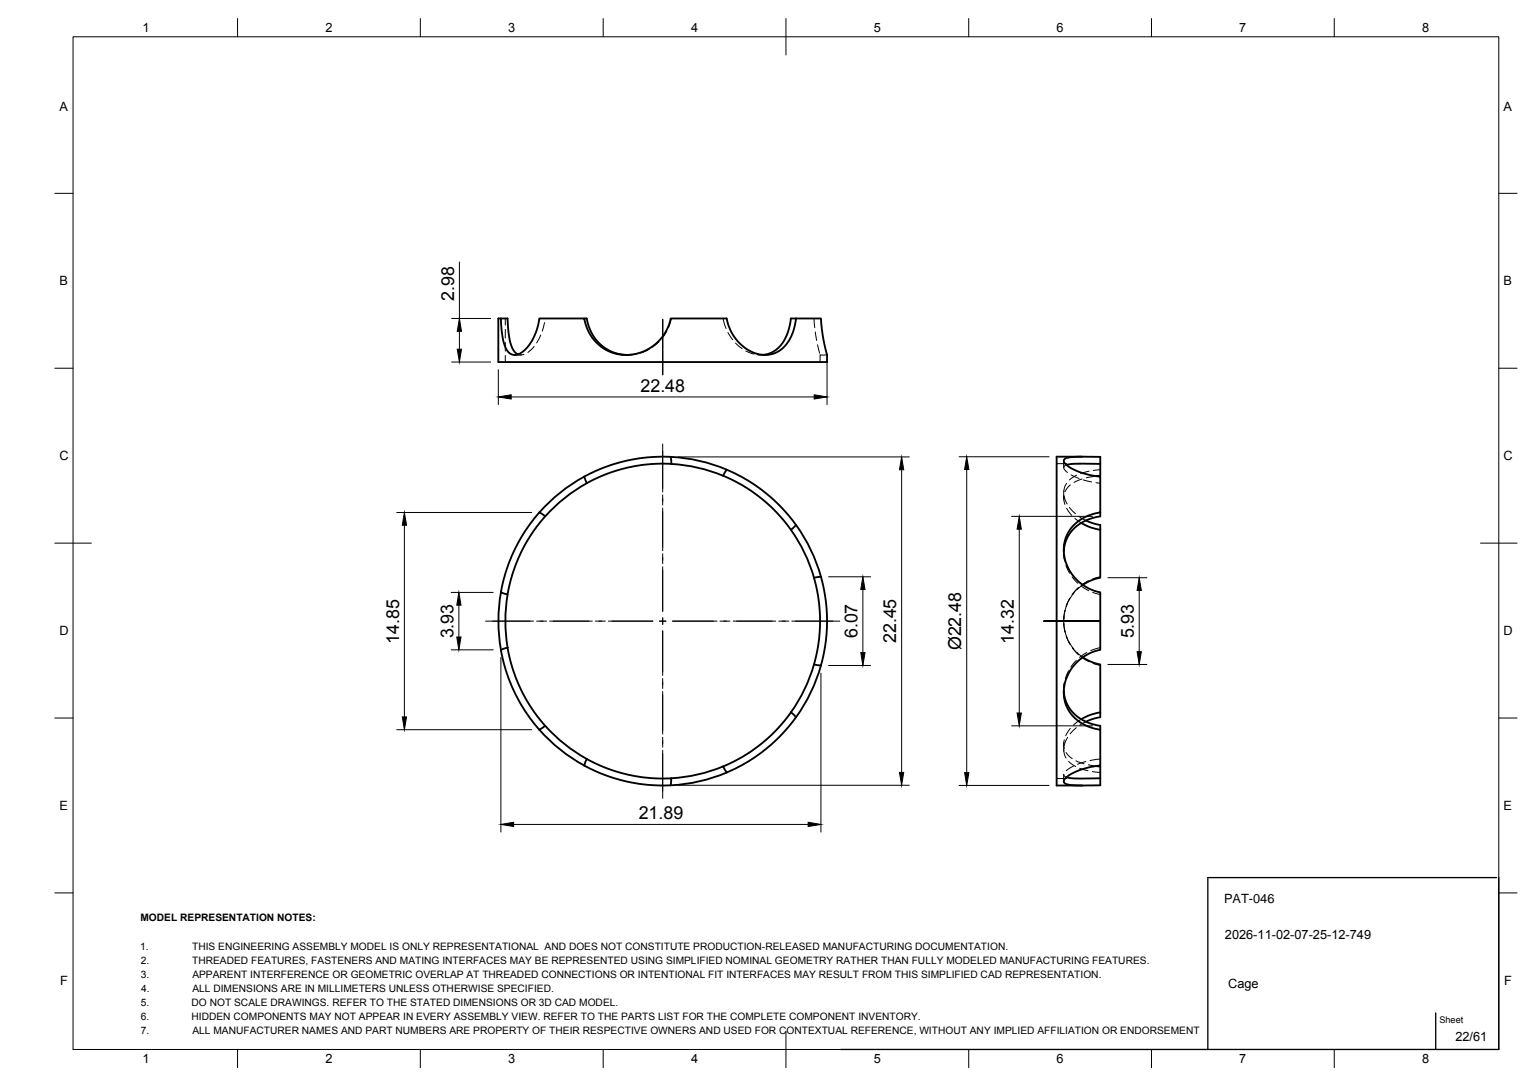
ISO-10303-21;
HEADER;
/* Generated by software containing ST-Developer
 * from STEP Tools, Inc. (www.steptools.com) 
 */

FILE_DESCRIPTION(
/* description */ ('Gear mesh backlash fixture'),
/* implementation_level */ '2;1');

FILE_NAME(
/* name */ 'Cage.step',
/* time_stamp */ '2026-10-28T03:26:00-07:00',
/* author */ (''),
/* organization */ (''),
/* preprocessor_version */ 'ST-DEVELOPER v20.2',
/* originating_system */ 'Autodesk Translation Framework v15.17.0.0',
/* authorisation */ '');

FILE_SCHEMA (('AUTOMOTIVE_DESIGN { 1 0 10303 214 3 1 1 }'));
ENDSEC;

DATA;
#10=MECHANICAL_DESIGN_GEOMETRIC_PRESENTATION_REPRESENTATION('',(#1037),#57900);
#736=SPHERICAL_SURFACE('',#14553,0.309556);
#737=SPHERICAL_SURFACE('',#14569,0.309556);
#738=SPHERICAL_SURFACE('',#14574,0.309556);
#739=SPHERICAL_SURFACE('',#14580,0.309556);
#740=SPHERICAL_SURFACE('',#14585,0.309556);
#741=SPHERICAL_SURFACE('',#14590,0.309556);
#742=SPHERICAL_SURFACE('',#14598,0.309556);
#791=B_SPLINE_CURVE_WITH_KNOTS('',3,(#20144,#20145,#20146,#20147,#20148,
#20149,#20150,#20151,#20152,#20153,#20154,#20155,#20156,#20157,#20158,#20159,
#20160,#20161,#20162,#20163,#20164,#20165),.UNSPECIFIED.,.F.,.F.,(4,2,2,
2,2,2,2,2,2,2,4),(0.0591825211272536,0.157966726598481,0.236950089897721,
0.315933453196962,0.391576304923761,0.46721915665056,0.54286200837736,0.618504860104159,
0.697488223403399,0.77647158670264,0.875255792173867),.UNSPECIFIED.);
#792=B_SPLINE_CURVE_WITH_KNOTS('',3,(#20169,#20170,#20171,#20172,#20173,
#20174,#20175,#20176,#20177,#20178,#20179,#20180,#20181,#20182,#20183,#20184,
#20185,#20186,#20187,#20188,#20189,#20190),.UNSPECIFIED.,.F.,.F.,(4,2,2,
2,2,2,2,2,2,2,4),(0.0581119756758434,0.106553146291161,0.213106292582322,
0.30849933801665,0.386091982889075,0.4636846277615,0.541277272633925,0.61886991750635,
0.714262962940678,0.820816109231839,0.869257279847157),.UNSPECIFIED.);
#793=B_SPLINE_CURVE_WITH_KNOTS('',3,(#20196,#20197,#20198,#20199,#20200,
#20201,#20202,#20203,#20204,#20205,#20206,#20207,#20208,#20209,#20210,#20211,
#20212,#20213,#20214,#20215,#20216,#20217),.UNSPECIFIED.,.F.,.F.,(4,2,2,
2,2,2,2,2,2,2,4),(0.0581119756758434,0.106553146291161,0.213106292582322,
0.30849933801665,0.386091982889075,0.4636846277615,0.541277272633925,0.61886991750635,
0.714262962940679,0.820816109231839,0.869257279847157),.UNSPECIFIED.);
#794=B_SPLINE_CURVE_WITH_KNOTS('',3,(#20221,#20222,#20223,#20224,#20225,
#20226,#20227,#20228,#20229,#20230,#20231,#20232,#20233,#20234,#20235,#20236,
#20237,#20238,#20239,#20240,#20241,#20242),.UNSPECIFIED.,.F.,.F.,(4,2,2,
2,2,2,2,2,2,2,4),(0.0581119756758433,0.106553146291161,0.213106292582322,
0.308499338016649,0.386091982889075,0.4636846277615,0.541277272633925,0.61886991750635,
0.714262962940678,0.820816109231839,0.869257279847157),.UNSPECIFIED.);
#795=B_SPLINE_CURVE_WITH_KNOTS('',3,(#20251,#20252,#20253,#20254,#20255,
#20256,#20257,#20258,#20259,#20260,#20261,#20262,#20263,#20264,#20265,#20266,
#20267,#20268,#20269,#20270,#20271,#20272),.UNSPECIFIED.,.F.,.F.,(4,2,2,
2,2,2,2,2,2,2,4),(0.0581119756758433,0.106553146291161,0.213106292582322,
0.30849933801665,0.386091982889075,0.4636846277615,0.541277272633925,0.61886991750635,
0.714262962940678,0.820816109231839,0.869257279847157),.UNSPECIFIED.);
#796=B_SPLINE_CURVE_WITH_KNOTS('',3,(#20276,#20277,#20278,#20279,#20280,
#20281,#20282,#20283,#20284,#20285,#20286,#20287,#20288,#20289,#20290,#20291,
#20292,#20293,#20294,#20295,#20296,#20297),.UNSPECIFIED.,.F.,.F.,(4,2,2,
2,2,2,2,2,2,2,4),(0.0581119756758434,0.106553146291161,0.213106292582322,
0.30849933801665,0.386091982889075,0.4636846277615,0.541277272633925,0.61886991750635,
0.714262962940678,0.820816109231839,0.869257279847157),.UNSPECIFIED.);
#797=B_SPLINE_CURVE_WITH_KNOTS('',3,(#20301,#20302,#20303,#20304,#20305,
#20306,#20307,#20308,#20309,#20310,#20311,#20312,#20313,#20314,#20315,#20316,
#20317,#20318,#20319,#20320,#20321,#20322),.UNSPECIFIED.,.F.,.F.,(4,2,2,
2,2,2,2,2,2,2,4),(0.0581119756758434,0.106553146291161,0.213106292582322,
0.30849933801665,0.386091982889075,0.4636846277615,0.541277272633925,0.61886991750635,
0.714262962940678,0.820816109231839,0.869257279847157),.UNSPECIFIED.);
#798=B_SPLINE_CURVE_WITH_KNOTS('',3,(#20326,#20327,#20328,#20329,#20330,
#20331,#20332,#20333,#20334,#20335,#20336,#20337,#20338,#20339,#20340,#20341,
#20342,#20343,#20344,#20345,#20346,#20347),.UNSPECIFIED.,.F.,.F.,(4,2,2,
2,2,2,2,2,2,2,4),(0.0581119756758433,0.106553146291161,0.213106292582322,
0.30849933801665,0.386091982889075,0.4636846277615,0.541277272633925,0.61886991750635,
0.714262962940678,0.820816109231839,0.869257279847157),.UNSPECIFIED.);
#799=B_SPLINE_CURVE_WITH_KNOTS('',3,(#20355,#20356,#20357,#20358,#20359,
#20360,#20361,#20362,#20363,#20364,#20365,#20366,#20367,#20368,#20369,#20370,
#20371,#20372,#20373,#20374,#20375,#20376),.UNSPECIFIED.,.F.,.F.,(4,2,2,
2,2,2,2,2,2,2,4),(0.0591825211272536,0.157966726598481,0.236950089897721,
0.315933453196962,0.391576304923761,0.467219156650561,0.54286200837736,
0.618504860104159,0.697488223403399,0.77647158670264,0.875255792173867),
 .UNSPECIFIED.);
#800=B_SPLINE_CURVE_WITH_KNOTS('',3,(#20384,#20385,#20386,#20387,#20388,
#20389,#20390,#20391,#20392,#20393,#20394,#20395,#20396,#20397,#20398,#20399,
#20400,#20401,#20402,#20403,#20404,#20405),.UNSPECIFIED.,.F.,.F.,(4,2,2,
2,2,2,2,2,2,2,4),(0.0591825211272536,0.157966726598481,0.236950089897722,
0.315933453196962,0.391576304923761,0.467219156650561,0.54286200837736,
0.618504860104159,0.697488223403399,0.77647158670264,0.875255792173867),
 .UNSPECIFIED.);
#801=B_SPLINE_CURVE_WITH_KNOTS('',3,(#20415,#20416,#20417,#20418,#20419,
#20420,#20421,#20422,#20423,#20424,#20425,#20426,#20427,#20428,#20429,#20430,
#20431,#20432,#20433,#20434,#20435,#20436),.UNSPECIFIED.,.F.,.F.,(4,2,2,
2,2,2,2,2,2,2,4),(0.0591825211272536,0.157966726598481,0.236950089897721,
0.315933453196962,0.391576304923761,0.46721915665056,0.54286200837736,0.618504860104159,
0.697488223403399,0.77647158670264,0.875255792173867),.UNSPECIFIED.);
#802=B_SPLINE_CURVE_WITH_KNOTS('',3,(#20444,#20445,#20446,#20447,#20448,
#20449,#20450,#20451,#20452,#20453,#20454,#20455,#20456,#20457,#20458,#20459,
#20460,#20461,#20462,#20463,#20464,#20465),.UNSPECIFIED.,.F.,.F.,(4,2,2,
2,2,2,2,2,2,2,4),(0.0591825211272536,0.157966726598481,0.236950089897721,
0.315933453196962,0.391576304923761,0.46721915665056,0.542862008377359,
0.618504860104159,0.697488223403399,0.776471586702639,0.875255792173867),
 .UNSPECIFIED.);
#803=B_SPLINE_CURVE_WITH_KNOTS('',3,(#20473,#20474,#20475,#20476,#20477,
#20478,#20479,#20480,#20481,#20482,#20483,#20484,#20485,#20486,#20487,#20488,
#20489,#20490,#20491,#20492,#20493,#20494),.UNSPECIFIED.,.F.,.F.,(4,2,2,
2,2,2,2,2,2,2,4),(0.0591825211272536,0.157966726598481,0.236950089897721,
0.315933453196962,0.391576304923761,0.46721915665056,0.54286200837736,0.618504860104159,
0.697488223403399,0.77647158670264,0.875255792173867),.UNSPECIFIED.);
#804=B_SPLINE_CURVE_WITH_KNOTS('',3,(#20503,#20504,#20505,#20506,#20507,
#20508,#20509,#20510,#20511,#20512,#20513,#20514,#20515,#20516,#20517,#20518,
#20519,#20520,#20521,#20522,#20523,#20524),.UNSPECIFIED.,.F.,.F.,(4,2,2,
2,2,2,2,2,2,2,4),(0.0591825211272536,0.157966726598481,0.236950089897721,
0.315933453196962,0.391576304923761,0.46721915665056,0.542862008377359,
0.618504860104159,0.697488223403399,0.776471586702639,0.875255792173867),
 .UNSPECIFIED.);
#931=SHAPE_REPRESENTATION_RELATIONSHIP('SRR','None',#58127,#981);
#981=ADVANCED_BREP_SHAPE_REPRESENTATION('',(#1102),#57860);
#1037=STYLED_ITEM('',(#58465),#1102);
#1102=MANIFOLD_SOLID_BREP('Continuous crown cage',#13597);
#1221=FACE_BOUND('',#2722,.T.);
#1417=PLANE('',#14566);
#1418=PLANE('',#14571);
#1419=PLANE('',#14576);
#1420=PLANE('',#14582);
#1421=PLANE('',#14587);
#1422=PLANE('',#14596);
#1423=PLANE('',#14600);
#1424=PLANE('',#14601);
#1863=FACE_OUTER_BOUND('',#2706,.T.);
#1864=FACE_OUTER_BOUND('',#2707,.T.);
#1865=FACE_OUTER_BOUND('',#2708,.T.);
#1866=FACE_OUTER_BOUND('',#2709,.T.);
#1867=FACE_OUTER_BOUND('',#2710,.T.);
#1868=FACE_OUTER_BOUND('',#2711,.T.);
#1869=FACE_OUTER_BOUND('',#2712,.T.);
#1870=FACE_OUTER_BOUND('',#2713,.T.);
#1871=FACE_OUTER_BOUND('',#2714,.T.);
#1872=FACE_OUTER_BOUND('',#2715,.T.);
#1873=FACE_OUTER_BOUND('',#2716,.T.);
#1874=FACE_OUTER_BOUND('',#2717,.T.);
#1875=FACE_OUTER_BOUND('',#2718,.T.);
#1876=FACE_OUTER_BOUND('',#2719,.T.);
#1877=FACE_OUTER_BOUND('',#2720,.T.);
#1878=FACE_OUTER_BOUND('',#2721,.T.);
#1879=FACE_OUTER_BOUND('',#2723,.T.);
#2706=EDGE_LOOP('',(#9625,#9626,#9627,#9628));
#2707=EDGE_LOOP('',(#9629,#9630,#9631,#9632,#9633,#9634,#9635,#9636,#9637,
#9638,#9639,#9640,#9641,#9642,#9643,#9644,#9645,#9646));
#2708=EDGE_LOOP('',(#9647,#9648,#9649,#9650));
#2709=EDGE_LOOP('',(#9651,#9652,#9653,#9654));
#2710=EDGE_LOOP('',(#9655,#9656,#9657,#9658));
#2711=EDGE_LOOP('',(#9659,#9660,#9661,#9662));
#2712=EDGE_LOOP('',(#9663,#9664,#9665,#9666,#9667,#9668));
#2713=EDGE_LOOP('',(#9669,#9670,#9671,#9672));
#2714=EDGE_LOOP('',(#9673,#9674,#9675,#9676));
#2715=EDGE_LOOP('',(#9677,#9678,#9679,#9680));
#2716=EDGE_LOOP('',(#9681,#9682,#9683,#9684));
#2717=EDGE_LOOP('',(#9685,#9686,#9687,#9688));
#2718=EDGE_LOOP('',(#9689,#9690,#9691,#9692,#9693,#9694,#9695,#9696,#9697,
#9698,#9699,#9700,#9701,#9702,#9703,#9704,#9705,#9706));
#2719=EDGE_LOOP('',(#9707,#9708,#9709,#9710));
#2720=EDGE_LOOP('',(#9711,#9712,#9713,#9714));
#2721=EDGE_LOOP('',(#9715));
#2722=EDGE_LOOP('',(#9716));
#2723=EDGE_LOOP('',(#9717,#9718,#9719,#9720));
#3607=LINE('',#20246,#4496);
#3608=LINE('',#20499,#4497);
#4496=VECTOR('',#16504,1.123812);
#4497=VECTOR('',#16573,1.076188);
#5359=CIRCLE('',#14554,0.303778037777585);
#5360=CIRCLE('',#14555,0.303778037777585);
#5361=CIRCLE('',#14557,1.123812);
#5362=CIRCLE('',#14558,1.123812);
#5363=CIRCLE('',#14559,1.123812);
#5364=CIRCLE('',#14560,1.123812);
#5365=CIRCLE('',#14561,1.123812);
#5366=CIRCLE('',#14562,1.123812);
#5367=CIRCLE('',#14563,1.123812);
#5368=CIRCLE('',#14564,1.123812);
#5369=CIRCLE('',#14565,1.123812);
#5370=CIRCLE('',#14567,1.076188);
#5371=CIRCLE('',#14568,0.303778037777585);
#5372=CIRCLE('',#14570,0.303778037777585);
#5373=CIRCLE('',#14572,1.076188);
#5374=CIRCLE('',#14573,0.303778037777585);
#5375=CIRCLE('',#14575,0.303778037777585);
#5376=CIRCLE('',#14577,1.076188);
#5377=CIRCLE('',#14578,1.076188);
#5378=CIRCLE('',#14579,0.303778037777585);
#5379=CIRCLE('',#14581,0.303778037777585);
#5380=CIRCLE('',#14583,1.076188);
#5381=CIRCLE('',#14584,0.303778037777585);
#5382=CIRCLE('',#14586,0.303778037777585);
#5383=CIRCLE('',#14588,1.076188);
#5384=CIRCLE('',#14589,0.303778037777585);
#5385=CIRCLE('',#14591,0.303778037777585);
#5386=CIRCLE('',#14593,1.076188);
#5387=CIRCLE('',#14594,1.076188);
#5388=CIRCLE('',#14595,1.076188);
#5389=CIRCLE('',#14597,0.303778037777585);
#5390=CIRCLE('',#14599,0.303778037777585);
#6033=VERTEX_POINT('',#20142);
#6034=VERTEX_POINT('',#20143);
#6035=VERTEX_POINT('',#20166);
#6036=VERTEX_POINT('',#20168);
#6037=VERTEX_POINT('',#20193);
#6038=VERTEX_POINT('',#20195);
#6039=VERTEX_POINT('',#20218);
#6040=VERTEX_POINT('',#20220);
#6041=VERTEX_POINT('',#20243);
#6042=VERTEX_POINT('',#20245);
#6043=VERTEX_POINT('',#20248);
#6044=VERTEX_POINT('',#20250);
#6045=VERTEX_POINT('',#20273);
#6046=VERTEX_POINT('',#20275);
#6047=VERTEX_POINT('',#20298);
#6048=VERTEX_POINT('',#20300);
#6049=VERTEX_POINT('',#20323);
#6050=VERTEX_POINT('',#20325);
#6051=VERTEX_POINT('',#20350);
#6052=VERTEX_POINT('',#20354);
#6053=VERTEX_POINT('',#20379);
#6054=VERTEX_POINT('',#20383);
#6055=VERTEX_POINT('',#20408);
#6056=VERTEX_POINT('',#20410);
#6057=VERTEX_POINT('',#20414);
#6058=VERTEX_POINT('',#20439);
#6059=VERTEX_POINT('',#20443);
#6060=VERTEX_POINT('',#20468);
#6061=VERTEX_POINT('',#20472);
#6062=VERTEX_POINT('',#20497);
#6063=VERTEX_POINT('',#20500);
#6064=VERTEX_POINT('',#20502);
#7399=EDGE_CURVE('',#6033,#6034,#791,.T.);
#7400=EDGE_CURVE('',#6035,#6033,#5359,.T.);
#7401=EDGE_CURVE('',#6036,#6035,#792,.T.);
#7402=EDGE_CURVE('',#6034,#6036,#5360,.T.);
#7403=EDGE_CURVE('',#6037,#6035,#5361,.T.);
#7404=EDGE_CURVE('',#6037,#6038,#793,.T.);
#7405=EDGE_CURVE('',#6039,#6038,#5362,.T.);
#7406=EDGE_CURVE('',#6039,#6040,#794,.T.);
#7407=EDGE_CURVE('',#6041,#6040,#5363,.T.);
#7408=EDGE_CURVE('',#6041,#6042,#3607,.T.);
#7409=EDGE_CURVE('',#6042,#6042,#5364,.T.);
#7410=EDGE_CURVE('',#6043,#6041,#5365,.T.);
#7411=EDGE_CURVE('',#6043,#6044,#795,.T.);
#7412=EDGE_CURVE('',#6045,#6044,#5366,.T.);
#7413=EDGE_CURVE('',#6045,#6046,#796,.T.);
#7414=EDGE_CURVE('',#6047,#6046,#5367,.T.);
#7415=EDGE_CURVE('',#6047,#6048,#797,.T.);
#7416=EDGE_CURVE('',#6049,#6048,#5368,.T.);
#7417=EDGE_CURVE('',#6049,#6050,#798,.T.);
#7418=EDGE_CURVE('',#6036,#6050,#5369,.T.);
#7419=EDGE_CURVE('',#6033,#6051,#5370,.T.);
#7420=EDGE_CURVE('',#6051,#6037,#5371,.T.);
#7421=EDGE_CURVE('',#6052,#6051,#799,.T.);
#7422=EDGE_CURVE('',#6038,#6052,#5372,.T.);
#7423=EDGE_CURVE('',#6052,#6053,#5373,.T.);
#7424=EDGE_CURVE('',#6053,#6039,#5374,.T.);
#7425=EDGE_CURVE('',#6054,#6053,#800,.T.);
#7426=EDGE_CURVE('',#6040,#6054,#5375,.T.);
#7427=EDGE_CURVE('',#6054,#6055,#5376,.T.);
#7428=EDGE_CURVE('',#6055,#6056,#5377,.T.);
#7429=EDGE_CURVE('',#6056,#6043,#5378,.T.);
#7430=EDGE_CURVE('',#6057,#6056,#801,.T.);
#7431=EDGE_CURVE('',#6044,#6057,#5379,.T.);
#7432=EDGE_CURVE('',#6057,#6058,#5380,.T.);
#7433=EDGE_CURVE('',#6058,#6045,#5381,.T.);
#7434=EDGE_CURVE('',#6059,#6058,#802,.T.);
#7435=EDGE_CURVE('',#6046,#6059,#5382,.T.);
#7436=EDGE_CURVE('',#6059,#6060,#5383,.T.);
#7437=EDGE_CURVE('',#6060,#6047,#5384,.T.);
#7438=EDGE_CURVE('',#6061,#6060,#803,.T.);
#7439=EDGE_CURVE('',#6048,#6061,#5385,.T.);
#7440=EDGE_CURVE('',#6062,#6062,#5386,.T.);
#7441=EDGE_CURVE('',#6062,#6055,#3608,.T.);
#7442=EDGE_CURVE('',#6063,#6034,#5387,.T.);
#7443=EDGE_CURVE('',#6063,#6064,#804,.T.);
#7444=EDGE_CURVE('',#6061,#6064,#5388,.T.);
#7445=EDGE_CURVE('',#6050,#6063,#5389,.T.);
#7446=EDGE_CURVE('',#6064,#6049,#5390,.T.);
#9625=ORIENTED_EDGE('',*,*,#7399,.F.);
#9626=ORIENTED_EDGE('',*,*,#7400,.F.);
#9627=ORIENTED_EDGE('',*,*,#7401,.F.);
#9628=ORIENTED_EDGE('',*,*,#7402,.F.);
#9629=ORIENTED_EDGE('',*,*,#7401,.T.);
#9630=ORIENTED_EDGE('',*,*,#7403,.F.);
#9631=ORIENTED_EDGE('',*,*,#7404,.T.);
#9632=ORIENTED_EDGE('',*,*,#7405,.F.);
#9633=ORIENTED_EDGE('',*,*,#7406,.T.);
#9634=ORIENTED_EDGE('',*,*,#7407,.F.);
#9635=ORIENTED_EDGE('',*,*,#7408,.T.);
#9636=ORIENTED_EDGE('',*,*,#7409,.F.);
#9637=ORIENTED_EDGE('',*,*,#7408,.F.);
#9638=ORIENTED_EDGE('',*,*,#7410,.F.);
#9639=ORIENTED_EDGE('',*,*,#7411,.T.);
#9640=ORIENTED_EDGE('',*,*,#7412,.F.);
#9641=ORIENTED_EDGE('',*,*,#7413,.T.);
#9642=ORIENTED_EDGE('',*,*,#7414,.F.);
#9643=ORIENTED_EDGE('',*,*,#7415,.T.);
#9644=ORIENTED_EDGE('',*,*,#7416,.F.);
#9645=ORIENTED_EDGE('',*,*,#7417,.T.);
#9646=ORIENTED_EDGE('',*,*,#7418,.F.);
#9647=ORIENTED_EDGE('',*,*,#7400,.T.);
#9648=ORIENTED_EDGE('',*,*,#7419,.T.);
#9649=ORIENTED_EDGE('',*,*,#7420,.T.);
#9650=ORIENTED_EDGE('',*,*,#7403,.T.);
#9651=ORIENTED_EDGE('',*,*,#7421,.F.);
#9652=ORIENTED_EDGE('',*,*,#7422,.F.);
#9653=ORIENTED_EDGE('',*,*,#7404,.F.);
#9654=ORIENTED_EDGE('',*,*,#7420,.F.);
#9655=ORIENTED_EDGE('',*,*,#7422,.T.);
#9656=ORIENTED_EDGE('',*,*,#7423,.T.);
#9657=ORIENTED_EDGE('',*,*,#7424,.T.);
#9658=ORIENTED_EDGE('',*,*,#7405,.T.);
#9659=ORIENTED_EDGE('',*,*,#7425,.F.);
#9660=ORIENTED_EDGE('',*,*,#7426,.F.);
#9661=ORIENTED_EDGE('',*,*,#7406,.F.);
#9662=ORIENTED_EDGE('',*,*,#7424,.F.);
#9663=ORIENTED_EDGE('',*,*,#7426,.T.);
#9664=ORIENTED_EDGE('',*,*,#7427,.T.);
#9665=ORIENTED_EDGE('',*,*,#7428,.T.);
#9666=ORIENTED_EDGE('',*,*,#7429,.T.);
#9667=ORIENTED_EDGE('',*,*,#7410,.T.);
#9668=ORIENTED_EDGE('',*,*,#7407,.T.);
#9669=ORIENTED_EDGE('',*,*,#7430,.F.);
#9670=ORIENTED_EDGE('',*,*,#7431,.F.);
#9671=ORIENTED_EDGE('',*,*,#7411,.F.);
#9672=ORIENTED_EDGE('',*,*,#7429,.F.);
#9673=ORIENTED_EDGE('',*,*,#7431,.T.);
#9674=ORIENTED_EDGE('',*,*,#7432,.T.);
#9675=ORIENTED_EDGE('',*,*,#7433,.T.);
#9676=ORIENTED_EDGE('',*,*,#7412,.T.);
#9677=ORIENTED_EDGE('',*,*,#7434,.F.);
#9678=ORIENTED_EDGE('',*,*,#7435,.F.);
#9679=ORIENTED_EDGE('',*,*,#7413,.F.);
#9680=ORIENTED_EDGE('',*,*,#7433,.F.);
#9681=ORIENTED_EDGE('',*,*,#7435,.T.);
#9682=ORIENTED_EDGE('',*,*,#7436,.T.);
#9683=ORIENTED_EDGE('',*,*,#7437,.T.);
#9684=ORIENTED_EDGE('',*,*,#7414,.T.);
#9685=ORIENTED_EDGE('',*,*,#7415,.F.);
#9686=ORIENTED_EDGE('',*,*,#7437,.F.);
#9687=ORIENTED_EDGE('',*,*,#7438,.F.);
#9688=ORIENTED_EDGE('',*,*,#7439,.F.);
#9689=ORIENTED_EDGE('',*,*,#7440,.F.);
#9690=ORIENTED_EDGE('',*,*,#7441,.T.);
#9691=ORIENTED_EDGE('',*,*,#7427,.F.);
#9692=ORIENTED_EDGE('',*,*,#7425,.T.);
#9693=ORIENTED_EDGE('',*,*,#7423,.F.);
#9694=ORIENTED_EDGE('',*,*,#7421,.T.);
#9695=ORIENTED_EDGE('',*,*,#7419,.F.);
#9696=ORIENTED_EDGE('',*,*,#7399,.T.);
#9697=ORIENTED_EDGE('',*,*,#7442,.F.);
#9698=ORIENTED_EDGE('',*,*,#7443,.T.);
#9699=ORIENTED_EDGE('',*,*,#7444,.F.);
#9700=ORIENTED_EDGE('',*,*,#7438,.T.);
#9701=ORIENTED_EDGE('',*,*,#7436,.F.);
#9702=ORIENTED_EDGE('',*,*,#7434,.T.);
#9703=ORIENTED_EDGE('',*,*,#7432,.F.);
#9704=ORIENTED_EDGE('',*,*,#7430,.T.);
#9705=ORIENTED_EDGE('',*,*,#7428,.F.);
#9706=ORIENTED_EDGE('',*,*,#7441,.F.);
#9707=ORIENTED_EDGE('',*,*,#7402,.T.);
#9708=ORIENTED_EDGE('',*,*,#7418,.T.);
#9709=ORIENTED_EDGE('',*,*,#7445,.T.);
#9710=ORIENTED_EDGE('',*,*,#7442,.T.);
#9711=ORIENTED_EDGE('',*,*,#7417,.F.);
#9712=ORIENTED_EDGE('',*,*,#7446,.F.);
#9713=ORIENTED_EDGE('',*,*,#7443,.F.);
#9714=ORIENTED_EDGE('',*,*,#7445,.F.);
#9715=ORIENTED_EDGE('',*,*,#7409,.T.);
#9716=ORIENTED_EDGE('',*,*,#7440,.T.);
#9717=ORIENTED_EDGE('',*,*,#7439,.T.);
#9718=ORIENTED_EDGE('',*,*,#7444,.T.);
#9719=ORIENTED_EDGE('',*,*,#7446,.T.);
#9720=ORIENTED_EDGE('',*,*,#7416,.T.);
#12654=CYLINDRICAL_SURFACE('',#14556,1.123812);
#12655=CYLINDRICAL_SURFACE('',#14592,1.076188);
#12980=ADVANCED_FACE('',(#1863),#736,.F.);
#12981=ADVANCED_FACE('',(#1864),#12654,.T.);
#12982=ADVANCED_FACE('',(#1865),#1417,.T.);
#12983=ADVANCED_FACE('',(#1866),#737,.F.);
#12984=ADVANCED_FACE('',(#1867),#1418,.T.);
#12985=ADVANCED_FACE('',(#1868),#738,.F.);
#12986=ADVANCED_FACE('',(#1869),#1419,.T.);
#12987=ADVANCED_FACE('',(#1870),#739,.F.);
#12988=ADVANCED_FACE('',(#1871),#1420,.T.);
#12989=ADVANCED_FACE('',(#1872),#740,.F.);
#12990=ADVANCED_FACE('',(#1873),#1421,.T.);
#12991=ADVANCED_FACE('',(#1874),#741,.F.);
#12992=ADVANCED_FACE('',(#1875),#12655,.F.);
#12993=ADVANCED_FACE('',(#1876),#1422,.T.);
#12994=ADVANCED_FACE('',(#1877),#742,.F.);
#12995=ADVANCED_FACE('',(#1878,#1221),#1423,.T.);
#12996=ADVANCED_FACE('',(#1879),#1424,.T.);
#13597=CLOSED_SHELL('',(#12980,#12981,#12982,#12983,#12984,#12985,#12986,
#12987,#12988,#12989,#12990,#12991,#12992,#12993,#12994,#12995,#12996));
#14552=AXIS2_PLACEMENT_3D('',#20140,#16488,#16489);
#14553=AXIS2_PLACEMENT_3D('',#20141,#16490,#16491);
#14554=AXIS2_PLACEMENT_3D('',#20167,#16492,#16493);
#14555=AXIS2_PLACEMENT_3D('',#20191,#16494,#16495);
#14556=AXIS2_PLACEMENT_3D('',#20192,#16496,#16497);
#14557=AXIS2_PLACEMENT_3D('',#20194,#16498,#16499);
#14558=AXIS2_PLACEMENT_3D('',#20219,#16500,#16501);
#14559=AXIS2_PLACEMENT_3D('',#20244,#16502,#16503);
#14560=AXIS2_PLACEMENT_3D('',#20247,#16505,#16506);
#14561=AXIS2_PLACEMENT_3D('',#20249,#16507,#16508);
#14562=AXIS2_PLACEMENT_3D('',#20274,#16509,#16510);
#14563=AXIS2_PLACEMENT_3D('',#20299,#16511,#16512);
#14564=AXIS2_PLACEMENT_3D('',#20324,#16513,#16514);
#14565=AXIS2_PLACEMENT_3D('',#20348,#16515,#16516);
#14566=AXIS2_PLACEMENT_3D('',#20349,#16517,#16518);
#14567=AXIS2_PLACEMENT_3D('',#20351,#16519,#16520);
#14568=AXIS2_PLACEMENT_3D('',#20352,#16521,#16522);
#14569=AXIS2_PLACEMENT_3D('',#20353,#16523,#16524);
#14570=AXIS2_PLACEMENT_3D('',#20377,#16525,#16526);
#14571=AXIS2_PLACEMENT_3D('',#20378,#16527,#16528);
#14572=AXIS2_PLACEMENT_3D('',#20380,#16529,#16530);
#14573=AXIS2_PLACEMENT_3D('',#20381,#16531,#16532);
#14574=AXIS2_PLACEMENT_3D('',#20382,#16533,#16534);
#14575=AXIS2_PLACEMENT_3D('',#20406,#16535,#16536);
#14576=AXIS2_PLACEMENT_3D('',#20407,#16537,#16538);
#14577=AXIS2_PLACEMENT_3D('',#20409,#16539,#16540);
#14578=AXIS2_PLACEMENT_3D('',#20411,#16541,#16542);
#14579=AXIS2_PLACEMENT_3D('',#20412,#16543,#16544);
#14580=AXIS2_PLACEMENT_3D('',#20413,#16545,#16546);
#14581=AXIS2_PLACEMENT_3D('',#20437,#16547,#16548);
#14582=AXIS2_PLACEMENT_3D('',#20438,#16549,#16550);
#14583=AXIS2_PLACEMENT_3D('',#20440,#16551,#16552);
#14584=AXIS2_PLACEMENT_3D('',#20441,#16553,#16554);
#14585=AXIS2_PLACEMENT_3D('',#20442,#16555,#16556);
#14586=AXIS2_PLACEMENT_3D('',#20466,#16557,#16558);
#14587=AXIS2_PLACEMENT_3D('',#20467,#16559,#16560);
#14588=AXIS2_PLACEMENT_3D('',#20469,#16561,#16562);
#14589=AXIS2_PLACEMENT_3D('',#20470,#16563,#16564);
#14590=AXIS2_PLACEMENT_3D('',#20471,#16565,#16566);
#14591=AXIS2_PLACEMENT_3D('',#20495,#16567,#16568);
#14592=AXIS2_PLACEMENT_3D('',#20496,#16569,#16570);
#14593=AXIS2_PLACEMENT_3D('',#20498,#16571,#16572);
#14594=AXIS2_PLACEMENT_3D('',#20501,#16574,#16575);
#14595=AXIS2_PLACEMENT_3D('',#20525,#16576,#16577);
#14596=AXIS2_PLACEMENT_3D('',#20526,#16578,#16579);
#14597=AXIS2_PLACEMENT_3D('',#20527,#16580,#16581);
#14598=AXIS2_PLACEMENT_3D('',#20528,#16582,#16583);
#14599=AXIS2_PLACEMENT_3D('',#20529,#16584,#16585);
#14600=AXIS2_PLACEMENT_3D('',#20530,#16586,#16587);
#14601=AXIS2_PLACEMENT_3D('',#20531,#16588,#16589);
#16488=DIRECTION('axis',(0.,0.,1.));
#16489=DIRECTION('refdir',(1.,0.,0.));
#16490=DIRECTION('center_axis',(0.,0.,1.));
#16491=DIRECTION('ref_axis',(1.,0.,0.));
#16492=DIRECTION('center_axis',(0.,-1.,0.));
#16493=DIRECTION('ref_axis',(0.,0.,-1.));
#16494=DIRECTION('center_axis',(0.,-1.,0.));
#16495=DIRECTION('ref_axis',(0.,0.,-1.));
#16496=DIRECTION('center_axis',(0.,1.,0.));
#16497=DIRECTION('ref_axis',(1.,0.,0.));
#16498=DIRECTION('center_axis',(0.,1.,0.));
#16499=DIRECTION('ref_axis',(1.,0.,0.));
#16500=DIRECTION('center_axis',(0.,1.,0.));
#16501=DIRECTION('ref_axis',(1.,0.,0.));
#16502=DIRECTION('center_axis',(0.,1.,0.));
#16503=DIRECTION('ref_axis',(1.,0.,0.));
#16504=DIRECTION('',(0.,-1.,0.));
#16505=DIRECTION('center_axis',(0.,-1.,0.));
#16506=DIRECTION('ref_axis',(1.,0.,0.));
#16507=DIRECTION('center_axis',(0.,1.,0.));
#16508=DIRECTION('ref_axis',(1.,0.,0.));
#16509=DIRECTION('center_axis',(0.,1.,0.));
#16510=DIRECTION('ref_axis',(1.,0.,0.));
#16511=DIRECTION('center_axis',(0.,1.,0.));
#16512=DIRECTION('ref_axis',(1.,0.,0.));
#16513=DIRECTION('center_axis',(0.,1.,0.));
#16514=DIRECTION('ref_axis',(1.,0.,0.));
#16515=DIRECTION('center_axis',(0.,1.,0.));
#16516=DIRECTION('ref_axis',(1.,0.,0.));
#16517=DIRECTION('center_axis',(0.,1.,0.));
#16518=DIRECTION('ref_axis',(1.,0.,0.));
#16519=DIRECTION('center_axis',(0.,-1.,0.));
#16520=DIRECTION('ref_axis',(1.,0.,0.));
#16521=DIRECTION('center_axis',(0.,-1.,0.));
#16522=DIRECTION('ref_axis',(0.,0.,-1.));
#16523=DIRECTION('center_axis',(8.96625347776458E-17,0.,1.));
#16524=DIRECTION('ref_axis',(1.,0.,0.));
#16525=DIRECTION('center_axis',(0.,-1.,0.));
#16526=DIRECTION('ref_axis',(0.,0.,-1.));
#16527=DIRECTION('center_axis',(0.,1.,0.));
#16528=DIRECTION('ref_axis',(1.,0.,0.));
#16529=DIRECTION('center_axis',(0.,-1.,0.));
#16530=DIRECTION('ref_axis',(1.,0.,0.));
#16531=DIRECTION('center_axis',(0.,-1.,0.));
#16532=DIRECTION('ref_axis',(0.,0.,-1.));
#16533=DIRECTION('center_axis',(0.,0.,1.));
#16534=DIRECTION('ref_axis',(1.,0.,0.));
#16535=DIRECTION('center_axis',(0.,-1.,0.));
#16536=DIRECTION('ref_axis',(0.,0.,-1.));
#16537=DIRECTION('center_axis',(0.,1.,0.));
#16538=DIRECTION('ref_axis',(1.,0.,0.));
#16539=DIRECTION('center_axis',(0.,-1.,0.));
#16540=DIRECTION('ref_axis',(1.,0.,0.));
#16541=DIRECTION('center_axis',(0.,-1.,0.));
#16542=DIRECTION('ref_axis',(1.,0.,0.));
#16543=DIRECTION('center_axis',(0.,-1.,0.));
#16544=DIRECTION('ref_axis',(0.,0.,-1.));
#16545=DIRECTION('center_axis',(0.,0.,1.));
#16546=DIRECTION('ref_axis',(1.,0.,0.));
#16547=DIRECTION('center_axis',(0.,-1.,0.));
#16548=DIRECTION('ref_axis',(0.,0.,-1.));
#16549=DIRECTION('center_axis',(0.,1.,0.));
#16550=DIRECTION('ref_axis',(1.,0.,0.));
#16551=DIRECTION('center_axis',(0.,-1.,0.));
#16552=DIRECTION('ref_axis',(1.,0.,0.));
#16553=DIRECTION('center_axis',(0.,-1.,0.));
#16554=DIRECTION('ref_axis',(0.,0.,-1.));
#16555=DIRECTION('center_axis',(8.96625347776458E-17,0.,1.));
#16556=DIRECTION('ref_axis',(1.,0.,0.));
#16557=DIRECTION('center_axis',(0.,-1.,0.));
#16558=DIRECTION('ref_axis',(0.,0.,-1.));
#16559=DIRECTION('center_axis',(0.,1.,0.));
#16560=DIRECTION('ref_axis',(1.,0.,0.));
#16561=DIRECTION('center_axis',(0.,-1.,0.));
#16562=DIRECTION('ref_axis',(1.,0.,0.));
#16563=DIRECTION('center_axis',(0.,-1.,0.));
#16564=DIRECTION('ref_axis',(0.,0.,-1.));
#16565=DIRECTION('center_axis',(0.,0.,1.));
#16566=DIRECTION('ref_axis',(1.,0.,0.));
#16567=DIRECTION('center_axis',(0.,-1.,0.));
#16568=DIRECTION('ref_axis',(0.,0.,-1.));
#16569=DIRECTION('center_axis',(0.,1.,0.));
#16570=DIRECTION('ref_axis',(1.,0.,0.));
#16571=DIRECTION('center_axis',(0.,1.,0.));
#16572=DIRECTION('ref_axis',(1.,0.,0.));
#16573=DIRECTION('',(0.,1.,0.));
#16574=DIRECTION('center_axis',(0.,-1.,0.));
#16575=DIRECTION('ref_axis',(1.,0.,0.));
#16576=DIRECTION('center_axis',(0.,-1.,0.));
#16577=DIRECTION('ref_axis',(1.,0.,0.));
#16578=DIRECTION('center_axis',(0.,1.,0.));
#16579=DIRECTION('ref_axis',(1.,0.,0.));
#16580=DIRECTION('center_axis',(0.,-1.,0.));
#16581=DIRECTION('ref_axis',(0.,0.,-1.));
#16582=DIRECTION('center_axis',(0.,0.,1.));
#16583=DIRECTION('ref_axis',(1.,0.,0.));
#16584=DIRECTION('center_axis',(0.,-1.,0.));
#16585=DIRECTION('ref_axis',(0.,0.,-1.));
#16586=DIRECTION('center_axis',(0.,-1.,0.));
#16587=DIRECTION('ref_axis',(-1.,0.,0.));
#16588=DIRECTION('center_axis',(0.,1.,0.));
#16589=DIRECTION('ref_axis',(1.,0.,0.));
#20140=CARTESIAN_POINT('',(0.,0.,0.));
#20141=CARTESIAN_POINT('Origin',(0.685838782044607,0.,0.860014630714833));
#20142=CARTESIAN_POINT('',(0.413083465285518,-0.05953,0.993751811093549));
#20143=CARTESIAN_POINT('',(0.876916659919095,-0.05953,0.623857181492959));
#20144=CARTESIAN_POINT('Ctrl Pts',(0.413083465285518,-0.05953,0.993751811093549));
#20145=CARTESIAN_POINT('Ctrl Pts',(0.419070565453383,-0.0925528133349865,
0.991263089003441));
#20146=CARTESIAN_POINT('Ctrl Pts',(0.430199341854858,-0.124911173756694,
0.986608710139579));
#20147=CARTESIAN_POINT('Ctrl Pts',(0.457978755888596,-0.177924977804098,
0.973971221090534));
#20148=CARTESIAN_POINT('Ctrl Pts',(0.473077587363685,-0.199697230012983,
0.966820759530997));
#20149=CARTESIAN_POINT('Ctrl Pts',(0.507057380724533,-0.237895043532788,
0.949440676105255));
#20150=CARTESIAN_POINT('Ctrl Pts',(0.525933334162555,-0.254319232363049,
0.939198248544428));
#20151=CARTESIAN_POINT('Ctrl Pts',(0.564362943424238,-0.28018331644634,
0.916597376014514));
#20152=CARTESIAN_POINT('Ctrl Pts',(0.585840553788742,-0.29104845371857,
0.903141581680914));
#20153=CARTESIAN_POINT('Ctrl Pts',(0.629305439856167,-0.30527573347708,
0.873412008702649));
#20154=CARTESIAN_POINT('Ctrl Pts',(0.651278921914856,-0.308638795020976,
0.857118508332695));
#20155=CARTESIAN_POINT('Ctrl Pts',(0.690705563850638,-0.308638795020976,
0.825676810575914));
#20156=CARTESIAN_POINT('Ctrl Pts',(0.711480111898423,-0.30527573347708,
0.807879894508811));
#20157=CARTESIAN_POINT('Ctrl Pts',(0.750136149454208,-0.29104845371857,
0.772120216227122));
#20158=CARTESIAN_POINT('Ctrl Pts',(0.768033796848072,-0.28018331644634,
0.754175290318038));
#20159=CARTESIAN_POINT('Ctrl Pts',(0.798619410861634,-0.254319232363049,
0.721738358858166));
#20160=CARTESIAN_POINT('Ctrl Pts',(0.812805334167529,-0.237895043532788,
0.705614819529209));
#20161=CARTESIAN_POINT('Ctrl Pts',(0.837310877969633,-0.199697230012983,
0.676354402927683));
#20162=CARTESIAN_POINT('Ctrl Pts',(0.847641868610495,-0.177924977804098,
0.663225258065736));
#20163=CARTESIAN_POINT('Ctrl Pts',(0.866144010579847,-0.124911173756694,
0.638954437806245));
#20164=CARTESIAN_POINT('Ctrl Pts',(0.873158080166742,-0.0925528133349865,
0.62914037979579));
#20165=CARTESIAN_POINT('Ctrl Pts',(0.876916659919095,-0.05953,0.623857181492959));
#20166=CARTESIAN_POINT('',(0.437601487681057,-0.05953,1.03511272300331));
#20167=CARTESIAN_POINT('Origin',(0.685838782044607,-0.05953,0.860014630714833));
#20168=CARTESIAN_POINT('',(0.911784794170997,-0.05953,0.656964154625313));
#20169=CARTESIAN_POINT('Ctrl Pts',(0.911784794170998,-0.0595300000000001,
0.656964154625312));
#20170=CARTESIAN_POINT('Ctrl Pts',(0.909827729890942,-0.0762225747374255,
0.659680317203144));
#20171=CARTESIAN_POINT('Ctrl Pts',(0.907004864562642,-0.0928409665394228,
0.663576540841106));
#20172=CARTESIAN_POINT('Ctrl Pts',(0.895234408667242,-0.144299303100741,
0.679480524217551));
#20173=CARTESIAN_POINT('Ctrl Pts',(0.882797231409153,-0.177024326825049,
0.695831250979106));
#20174=CARTESIAN_POINT('Ctrl Pts',(0.854332839576145,-0.227269801620064,
0.73042219438957));
#20175=CARTESIAN_POINT('Ctrl Pts',(0.834863020612702,-0.251265615809407,
0.752807465209441));
#20176=CARTESIAN_POINT('Ctrl Pts',(0.800439809856111,-0.279889827963178,
0.789147407129766));
#20177=CARTESIAN_POINT('Ctrl Pts',(0.781998747691871,-0.290879136862659,
0.80756613568454));
#20178=CARTESIAN_POINT('Ctrl Pts',(0.742239891936898,-0.305251990234487,
0.844254137480382));
#20179=CARTESIAN_POINT('Ctrl Pts',(0.720906778729541,-0.308638795020976,
0.862505527716294));
#20180=CARTESIAN_POINT('Ctrl Pts',(0.680463863683392,-0.308638795020976,
0.894757676234429));
#20181=CARTESIAN_POINT('Ctrl Pts',(0.657923009631182,-0.305251990234488,
0.91149460735272));
#20182=CARTESIAN_POINT('Ctrl Pts',(0.613307674922609,-0.290879136862659,
0.942092777160053));
#20183=CARTESIAN_POINT('Ctrl Pts',(0.591247219971725,-0.279889827963178,
0.955972930713954));
#20184=CARTESIAN_POINT('Ctrl Pts',(0.548158511259202,-0.251265615809407,
0.981446681891443));
#20185=CARTESIAN_POINT('Ctrl Pts',(0.522002043615455,-0.227269801620063,
0.995447160474328));
#20186=CARTESIAN_POINT('Ctrl Pts',(0.481944444320713,-0.177024326825049,
1.01550068154148));
#20187=CARTESIAN_POINT('Ctrl Pts',(0.463236132117164,-0.14429930310074,
1.0239876538093));
#20188=CARTESIAN_POINT('Ctrl Pts',(0.445111721969657,-0.0928409665394226,
1.03192403056628));
#20189=CARTESIAN_POINT('Ctrl Pts',(0.440685038163619,-0.0762225747374254,
1.03380912944435));
#20190=CARTESIAN_POINT('Ctrl Pts',(0.437601487681056,-0.05953,1.03511272300331));
#20191=CARTESIAN_POINT('Origin',(0.685838782044607,-0.05953,0.860014630714833));
#20192=CARTESIAN_POINT('Origin',(0.,-0.208355,0.));
#20193=CARTESIAN_POINT('',(0.0548532617164168,-0.05953,1.12247250791415));
#20194=CARTESIAN_POINT('Origin',(0.,-0.05953,0.));
#20195=CARTESIAN_POINT('',(-0.536443649899848,-0.05953,0.987512846410683));
#20196=CARTESIAN_POINT('Ctrl Pts',(0.0548532617164173,-0.0595300000000001,
1.12247250791414));
#20197=CARTESIAN_POINT('Ctrl Pts',(0.05150947068137,-0.0762225747374254,
1.12263591311425));
#20198=CARTESIAN_POINT('Ctrl Pts',(0.0467032526342597,-0.0928409665394227,
1.12285816383385));
#20199=CARTESIAN_POINT('Ctrl Pts',(0.0269302585198975,-0.144299303100741,
1.12357162229597));
#20200=CARTESIAN_POINT('Ctrl Pts',(0.006392292392153,-0.177024326825049,
1.12404235695137));
#20201=CARTESIAN_POINT('Ctrl Pts',(-0.0383992541984087,-0.227269801620063,
1.12335509974011));
#20202=CARTESIAN_POINT('Ctrl Pts',(-0.0680399972366993,-0.251265615809407,
1.12208997038458));
#20203=CARTESIAN_POINT('Ctrl Pts',(-0.117914228755037,-0.279889827963178,
1.1178344036749));
#20204=CARTESIAN_POINT('Ctrl Pts',(-0.14381238480104,-0.290879136862659,
1.11490049012186));
#20205=CARTESIAN_POINT('Ctrl Pts',(-0.19728546073067,-0.305251990234488,
1.10669035995599));
#20206=CARTESIAN_POINT('Ctrl Pts',(-0.224855950742601,-0.308638795020976,
1.10139101611326));
#20207=CARTESIAN_POINT('Ctrl Pts',(-0.275287440920027,-0.308638795020976,
1.0898803575765));
#20208=CARTESIAN_POINT('Ctrl Pts',(-0.302426893214945,-0.305251990234488,
1.08269251410343));
#20209=CARTESIAN_POINT('Ctrl Pts',(-0.35416671187353,-0.290879136862659,
1.06688848765783));
#20210=CARTESIAN_POINT('Ctrl Pts',(-0.3787731215897,-0.279889827963178,
1.05829506364875));
#20211=CARTESIAN_POINT('Ctrl Pts',(-0.425554672694338,-0.251265615809407,
1.04048957871266));
#20212=CARTESIAN_POINT('Ctrl Pts',(-0.452808978448581,-0.227269801620063,
1.02876878445619));
#20213=CARTESIAN_POINT('Ctrl Pts',(-0.493462957200432,-0.177024326825049,
1.0099536580922));
#20214=CARTESIAN_POINT('Ctrl Pts',(-0.511762781179148,-0.14429930310074,
1.00061845128527));
#20215=CARTESIAN_POINT('Ctrl Pts',(-0.529268075276157,-0.0928409665394226,
0.991396466802468));
#20216=CARTESIAN_POINT('Ctrl Pts',(-0.533501897135713,-0.0762225747374254,
0.989110885965947));
#20217=CARTESIAN_POINT('Ctrl Pts',(-0.536443649899848,-0.0595300000000001,
0.987512846410683));
#20218=CARTESIAN_POINT('',(-0.843383895613249,-0.05953,0.742736168477219));
#20219=CARTESIAN_POINT('Origin',(0.,-0.05953,0.));
#20220=CARTESIAN_POINT('',(-1.10653577764992,-0.05953,0.196295654879792));
#20221=CARTESIAN_POINT('Ctrl Pts',(-0.843383895613249,-0.0595300000000001,
0.742736168477219));
#20222=CARTESIAN_POINT('Ctrl Pts',(-0.84559647055299,-0.0762225747374255,
0.740223768851062));
#20223=CARTESIAN_POINT('Ctrl Pts',(-0.848766861100456,-0.0928409665394227,
0.736604687327351));
#20224=CARTESIAN_POINT('Ctrl Pts',(-0.861652925570091,-0.144299303100741,
0.721590372101268));
#20225=CARTESIAN_POINT('Ctrl Pts',(-0.87482617317514,-0.177024326825049,
0.705826641853758));
#20226=CARTESIAN_POINT('Ctrl Pts',(-0.902215926359523,-0.227269801620063,
0.670378702718353));
#20227=CARTESIAN_POINT('Ctrl Pts',(-0.919707509403859,-0.251265615809407,
0.646415841396062));
#20228=CARTESIAN_POINT('Ctrl Pts',(-0.947476448101718,-0.279889827963178,
0.604769294586516));
#20229=CARTESIAN_POINT('Ctrl Pts',(-0.961329858300736,-0.290879136862659,
0.582692035672022));
#20230=CARTESIAN_POINT('Ctrl Pts',(-0.988250837578047,-0.305251990234488,
0.535766169015486));
#20231=CARTESIAN_POINT('Ctrl Pts',(-1.00129756308006,-0.308638795020976,
0.510906605094603));
#20232=CARTESIAN_POINT('Ctrl Pts',(-1.02374168767024,-0.308638795020976,
0.46430090015576));
#20233=CARTESIAN_POINT('Ctrl Pts',(-1.03504317708586,-0.305251990234488,
0.438600874831839));
#20234=CARTESIAN_POINT('Ctrl Pts',(-1.05494634094458,-0.290879136862659,
0.388295406390235));
#20235=CARTESIAN_POINT('Ctrl Pts',(-1.06356957703048,-0.279889827963178,
0.363699428370917));
#20236=CARTESIAN_POINT('Ctrl Pts',(-1.0788165083757,-0.251265615809407,
0.316022600643821));
#20237=CARTESIAN_POINT('Ctrl Pts',(-1.08664560412098,-0.227269801620063,
0.287406530683752));
#20238=CARTESIAN_POINT('Ctrl Pts',(-1.09728268713976,-0.177024326825049,
0.243890930799337));
#20239=CARTESIAN_POINT('Ctrl Pts',(-1.10139388218929,-0.144299303100741,
0.22376314604679));
#20240=CARTESIAN_POINT('Ctrl Pts',(-1.10509821673782,-0.0928409665394227,
0.204327142733961));
#20241=CARTESIAN_POINT('Ctrl Pts',(-1.10595102243643,-0.0762225747374254,
0.199591971170104));
#20242=CARTESIAN_POINT('Ctrl Pts',(-1.10653577764992,-0.0595300000000001,
0.196295654879792));
#20243=CARTESIAN_POINT('',(-1.123812,-0.05953,1.37627276864339E-16));
#20244=CARTESIAN_POINT('Origin',(0.,-0.05953,0.));
#20245=CARTESIAN_POINT('',(-1.123812,-0.35718,1.37627276864339E-16));
#20246=CARTESIAN_POINT('',(-1.123812,-0.208355,1.37627276864339E-16));
#20247=CARTESIAN_POINT('Origin',(0.,-0.35718,0.));
#20248=CARTESIAN_POINT('',(-1.10653577764992,-0.05953,-0.196295654879793));
#20249=CARTESIAN_POINT('Origin',(0.,-0.05953,0.));
#20250=CARTESIAN_POINT('',(-0.843383895613249,-0.05953,-0.742736168477219));
#20251=CARTESIAN_POINT('Ctrl Pts',(-1.10653577764992,-0.0595300000000001,
-0.196295654879792));
#20252=CARTESIAN_POINT('Ctrl Pts',(-1.10595102243643,-0.0762225747374255,
-0.199591971170104));
#20253=CARTESIAN_POINT('Ctrl Pts',(-1.10509821673782,-0.0928409665394228,
-0.204327142733962));
#20254=CARTESIAN_POINT('Ctrl Pts',(-1.10139388218929,-0.144299303100741,
-0.22376314604679));
#20255=CARTESIAN_POINT('Ctrl Pts',(-1.09728268713976,-0.177024326825049,
-0.243890930799338));
#20256=CARTESIAN_POINT('Ctrl Pts',(-1.08664560412098,-0.227269801620063,
-0.287406530683753));
#20257=CARTESIAN_POINT('Ctrl Pts',(-1.0788165083757,-0.251265615809407,
-0.316022600643821));
#20258=CARTESIAN_POINT('Ctrl Pts',(-1.06356957703048,-0.279889827963178,
-0.363699428370918));
#20259=CARTESIAN_POINT('Ctrl Pts',(-1.05494634094458,-0.290879136862659,
-0.388295406390235));
#20260=CARTESIAN_POINT('Ctrl Pts',(-1.03504317708586,-0.305251990234488,
-0.438600874831839));
#20261=CARTESIAN_POINT('Ctrl Pts',(-1.02374168767024,-0.308638795020976,
-0.46430090015576));
#20262=CARTESIAN_POINT('Ctrl Pts',(-1.00129756308006,-0.308638795020976,
-0.510906605094603));
#20263=CARTESIAN_POINT('Ctrl Pts',(-0.988250837578047,-0.305251990234488,
-0.535766169015486));
#20264=CARTESIAN_POINT('Ctrl Pts',(-0.961329858300736,-0.290879136862659,
-0.582692035672022));
#20265=CARTESIAN_POINT('Ctrl Pts',(-0.947476448101718,-0.279889827963178,
-0.604769294586516));
#20266=CARTESIAN_POINT('Ctrl Pts',(-0.919707509403859,-0.251265615809407,
-0.646415841396062));
#20267=CARTESIAN_POINT('Ctrl Pts',(-0.902215926359523,-0.227269801620064,
-0.670378702718353));
#20268=CARTESIAN_POINT('Ctrl Pts',(-0.87482617317514,-0.177024326825049,
-0.705826641853758));
#20269=CARTESIAN_POINT('Ctrl Pts',(-0.861652925570091,-0.144299303100741,
-0.721590372101268));
#20270=CARTESIAN_POINT('Ctrl Pts',(-0.848766861100456,-0.0928409665394229,
-0.736604687327351));
#20271=CARTESIAN_POINT('Ctrl Pts',(-0.84559647055299,-0.0762225747374255,
-0.740223768851063));
#20272=CARTESIAN_POINT('Ctrl Pts',(-0.843383895613249,-0.0595300000000001,
-0.742736168477219));
#20273=CARTESIAN_POINT('',(-0.536443649899847,-0.05953,-0.987512846410683));
#20274=CARTESIAN_POINT('Origin',(0.,-0.05953,0.));
#20275=CARTESIAN_POINT('',(0.0548532617164172,-0.05953,-1.12247250791415));
#20276=CARTESIAN_POINT('Ctrl Pts',(-0.536443649899848,-0.0595300000000001,
-0.987512846410683));
#20277=CARTESIAN_POINT('Ctrl Pts',(-0.533501897135712,-0.0762225747374254,
-0.989110885965947));
#20278=CARTESIAN_POINT('Ctrl Pts',(-0.529268075276156,-0.0928409665394227,
-0.991396466802469));
#20279=CARTESIAN_POINT('Ctrl Pts',(-0.511762781179147,-0.144299303100741,
-1.00061845128527));
#20280=CARTESIAN_POINT('Ctrl Pts',(-0.493462957200432,-0.177024326825049,
-1.0099536580922));
#20281=CARTESIAN_POINT('Ctrl Pts',(-0.45280897844858,-0.227269801620063,
-1.02876878445619));
#20282=CARTESIAN_POINT('Ctrl Pts',(-0.425554672694337,-0.251265615809407,
-1.04048957871266));
#20283=CARTESIAN_POINT('Ctrl Pts',(-0.3787731215897,-0.279889827963178,
-1.05829506364875));
#20284=CARTESIAN_POINT('Ctrl Pts',(-0.354166711873529,-0.290879136862659,
-1.06688848765783));
#20285=CARTESIAN_POINT('Ctrl Pts',(-0.302426893214944,-0.305251990234488,
-1.08269251410343));
#20286=CARTESIAN_POINT('Ctrl Pts',(-0.275287440920027,-0.308638795020976,
-1.0898803575765));
#20287=CARTESIAN_POINT('Ctrl Pts',(-0.224855950742601,-0.308638795020976,
-1.10139101611326));
#20288=CARTESIAN_POINT('Ctrl Pts',(-0.19728546073067,-0.305251990234488,
-1.10669035995599));
#20289=CARTESIAN_POINT('Ctrl Pts',(-0.143812384801039,-0.290879136862659,
-1.11490049012186));
#20290=CARTESIAN_POINT('Ctrl Pts',(-0.117914228755037,-0.279889827963178,
-1.1178344036749));
#20291=CARTESIAN_POINT('Ctrl Pts',(-0.0680399972366989,-0.251265615809407,
-1.12208997038458));
#20292=CARTESIAN_POINT('Ctrl Pts',(-0.0383992541984084,-0.227269801620063,
-1.12335509974011));
#20293=CARTESIAN_POINT('Ctrl Pts',(0.00639229239215326,-0.177024326825049,
-1.12404235695137));
#20294=CARTESIAN_POINT('Ctrl Pts',(0.0269302585198977,-0.144299303100741,
-1.12357162229597));
#20295=CARTESIAN_POINT('Ctrl Pts',(0.04670325263426,-0.0928409665394228,
-1.12285816383385));
#20296=CARTESIAN_POINT('Ctrl Pts',(0.0515094706813703,-0.0762225747374255,
-1.12263591311425));
#20297=CARTESIAN_POINT('Ctrl Pts',(0.0548532617164176,-0.0595300000000001,
-1.12247250791414));
#20298=CARTESIAN_POINT('',(0.437601487681057,-0.05953,-1.03511272300331));
#20299=CARTESIAN_POINT('Origin',(0.,-0.05953,0.));
#20300=CARTESIAN_POINT('',(0.911784794170997,-0.05953,-0.656964154625313));
#20301=CARTESIAN_POINT('Ctrl Pts',(0.437601487681056,-0.0595300000000001,
-1.03511272300331));
#20302=CARTESIAN_POINT('Ctrl Pts',(0.440685038163619,-0.0762225747374255,
-1.03380912944435));
#20303=CARTESIAN_POINT('Ctrl Pts',(0.445111721969657,-0.0928409665394228,
-1.03192403056628));
#20304=CARTESIAN_POINT('Ctrl Pts',(0.463236132117164,-0.144299303100741,
-1.0239876538093));
#20305=CARTESIAN_POINT('Ctrl Pts',(0.481944444320713,-0.177024326825049,
-1.01550068154148));
#20306=CARTESIAN_POINT('Ctrl Pts',(0.522002043615455,-0.227269801620064,
-0.995447160474328));
#20307=CARTESIAN_POINT('Ctrl Pts',(0.548158511259203,-0.251265615809407,
-0.981446681891443));
#20308=CARTESIAN_POINT('Ctrl Pts',(0.591247219971725,-0.279889827963178,
-0.955972930713954));
#20309=CARTESIAN_POINT('Ctrl Pts',(0.613307674922609,-0.290879136862659,
-0.942092777160053));
#20310=CARTESIAN_POINT('Ctrl Pts',(0.657923009631182,-0.305251990234487,
-0.91149460735272));
#20311=CARTESIAN_POINT('Ctrl Pts',(0.680463863683393,-0.308638795020976,
-0.894757676234429));
#20312=CARTESIAN_POINT('Ctrl Pts',(0.720906778729542,-0.308638795020976,
-0.862505527716294));
#20313=CARTESIAN_POINT('Ctrl Pts',(0.742239891936899,-0.305251990234488,
-0.844254137480381));
#20314=CARTESIAN_POINT('Ctrl Pts',(0.781998747691872,-0.290879136862659,
-0.80756613568454));
#20315=CARTESIAN_POINT('Ctrl Pts',(0.800439809856112,-0.279889827963178,
-0.789147407129765));
#20316=CARTESIAN_POINT('Ctrl Pts',(0.834863020612702,-0.251265615809407,
-0.752807465209441));
#20317=CARTESIAN_POINT('Ctrl Pts',(0.854332839576145,-0.227269801620064,
-0.73042219438957));
#20318=CARTESIAN_POINT('Ctrl Pts',(0.882797231409153,-0.177024326825049,
-0.695831250979106));
#20319=CARTESIAN_POINT('Ctrl Pts',(0.895234408667242,-0.144299303100741,
-0.679480524217551));
#20320=CARTESIAN_POINT('Ctrl Pts',(0.907004864562642,-0.0928409665394228,
-0.663576540841106));
#20321=CARTESIAN_POINT('Ctrl Pts',(0.909827729890942,-0.0762225747374256,
-0.659680317203144));
#20322=CARTESIAN_POINT('Ctrl Pts',(0.911784794170998,-0.0595300000000001,
-0.656964154625312));
#20323=CARTESIAN_POINT('',(1.08212377959455,-0.05953,-0.303251606722892));
#20324=CARTESIAN_POINT('Origin',(0.,-0.05953,0.));
#20325=CARTESIAN_POINT('',(1.08212377959455,-0.05953,0.303251606722892));
#20326=CARTESIAN_POINT('Ctrl Pts',(1.08212377959455,-0.0595300000000001,
-0.303251606722892));
#20327=CARTESIAN_POINT('Ctrl Pts',(1.0830271513892,-0.0762225747374255,
-0.300028012588062));
#20328=CARTESIAN_POINT('Ctrl Pts',(1.08431331394788,-0.0928409665394228,
-0.2953917518996));
#20329=CARTESIAN_POINT('Ctrl Pts',(1.08940878963422,-0.144299303100741,
-0.276273267473431));
#20330=CARTESIAN_POINT('Ctrl Pts',(1.09443784939331,-0.177024326825049,
-0.256354979351213));
#20331=CARTESIAN_POINT('Ctrl Pts',(1.10373487993589,-0.227269801620064,
-0.212533521233765));
#20332=CARTESIAN_POINT('Ctrl Pts',(1.10909715583869,-0.251265615809407,
-0.183354415742157));
#20333=CARTESIAN_POINT('Ctrl Pts',(1.1160463456491,-0.279889827963178,-0.133783682657561));
#20334=CARTESIAN_POINT('Ctrl Pts',(1.11894887330541,-0.290879136862659,
-0.107881990270302));
#20335=CARTESIAN_POINT('Ctrl Pts',(1.12284346704144,-0.305251990234488,
-0.0539226701638766));
#20336=CARTESIAN_POINT('Ctrl Pts',(1.123812,-0.308638795020976,-0.025864214957475));
#20337=CARTESIAN_POINT('Ctrl Pts',(1.123812,-0.308638795020976,0.025864214957475));
#20338=CARTESIAN_POINT('Ctrl Pts',(1.12284346704144,-0.305251990234488,
0.0539226701638766));
#20339=CARTESIAN_POINT('Ctrl Pts',(1.11894887330541,-0.290879136862659,
0.107881990270302));
#20340=CARTESIAN_POINT('Ctrl Pts',(1.1160463456491,-0.279889827963178,0.133783682657561));
#20341=CARTESIAN_POINT('Ctrl Pts',(1.10909715583869,-0.251265615809407,
0.183354415742157));
#20342=CARTESIAN_POINT('Ctrl Pts',(1.10373487993589,-0.227269801620064,
0.212533521233765));
#20343=CARTESIAN_POINT('Ctrl Pts',(1.09443784939331,-0.177024326825049,
0.256354979351213));
#20344=CARTESIAN_POINT('Ctrl Pts',(1.08940878963422,-0.144299303100741,
0.276273267473431));
#20345=CARTESIAN_POINT('Ctrl Pts',(1.08431331394788,-0.0928409665394228,
0.2953917518996));
#20346=CARTESIAN_POINT('Ctrl Pts',(1.0830271513892,-0.0762225747374255,
0.300028012588062));
#20347=CARTESIAN_POINT('Ctrl Pts',(1.08212377959455,-0.0595300000000001,
0.303251606722892));
#20348=CARTESIAN_POINT('Origin',(0.,-0.05953,0.));
#20349=CARTESIAN_POINT('Origin',(0.,-0.05953,0.));
#20350=CARTESIAN_POINT('',(0.0589974094846122,-0.05953,1.07456964270265));
#20351=CARTESIAN_POINT('Origin',(0.,-0.05953,0.));
#20352=CARTESIAN_POINT('Origin',(-0.244773027351946,-0.05953,1.07242070340001));
#20353=CARTESIAN_POINT('Origin',(-0.244773027351946,0.,1.07242070340001));
#20354=CARTESIAN_POINT('',(-0.519393123750572,-0.05953,0.942555777842682));
#20355=CARTESIAN_POINT('Ctrl Pts',(-0.519393123750572,-0.05953,0.942555777842682));
#20356=CARTESIAN_POINT('Ctrl Pts',(-0.513714466572041,-0.0925528133349865,
0.945684988399766));
#20357=CARTESIAN_POINT('Ctrl Pts',(-0.503136848051455,-0.124911173756694,
0.951483858396181));
#20358=CARTESIAN_POINT('Ctrl Pts',(-0.47593627990192,-0.177924977804098,
0.965323333309091));
#20359=CARTESIAN_POINT('Ctrl Pts',(-0.460931856495794,-0.199697230012983,
0.972669835243841));
#20360=CARTESIAN_POINT('Ctrl Pts',(-0.426157505475872,-0.237895043532788,
0.988400002689705));
#20361=CARTESIAN_POINT('Ctrl Pts',(-0.406380688682952,-0.254319232363049,
0.996771768218699));
#20362=CARTESIAN_POINT('Ctrl Pts',(-0.364750145543744,-0.28018331644634,
1.01272583306292));
#20363=CARTESIAN_POINT('Ctrl Pts',(-0.340838910881557,-0.29104845371857,
1.02112815447116));
#20364=CARTESIAN_POINT('Ctrl Pts',(-0.290495481564827,-0.30527573347708,
1.036574285215));
#20365=CARTESIAN_POINT('Ctrl Pts',(-0.264056468041074,-0.308638795020976,
1.04359501395068));
#20366=CARTESIAN_POINT('Ctrl Pts',(-0.214892249704082,-0.308638795020976,
1.05481642595959));
#20367=CARTESIAN_POINT('Ctrl Pts',(-0.188025341585962,-0.30527573347708,
1.05996242598502));
#20368=CARTESIAN_POINT('Ctrl Pts',(-0.135965654106109,-0.29104845371857,
1.06788913840721));
#20369=CARTESIAN_POINT('Ctrl Pts',(-0.110776745452494,-0.28018331644634,
1.07069360430242));
#20370=CARTESIAN_POINT('Ctrl Pts',(-0.0663467128214646,-0.254319232363049,
1.07438230428002));
#20371=CARTESIAN_POINT('Ctrl Pts',(-0.0448960436540983,-0.237895043532788,
1.07542044338697));
#20372=CARTESIAN_POINT('Ctrl Pts',(-0.00674037211528124,-0.199697230012983,
1.07633607767727));
#20373=CARTESIAN_POINT('Ctrl Pts',(0.00996567398334777,-0.177924977804098,
1.07622728347683));
#20374=CARTESIAN_POINT('Ctrl Pts',(0.0404772621979741,-0.124911173756694,
1.07556023164702));
#20375=CARTESIAN_POINT('Ctrl Pts',(0.0525234025782719,-0.0925528133349865,
1.07492508698591));
#20376=CARTESIAN_POINT('Ctrl Pts',(0.0589974094846124,-0.05953,1.07456964270265));
#20377=CARTESIAN_POINT('Origin',(-0.244773027351946,-0.05953,1.07242070340001));
#20378=CARTESIAN_POINT('Origin',(0.,-0.05953,0.));
#20379=CARTESIAN_POINT('',(-0.803348093619616,-0.05953,0.716109245731214));
#20380=CARTESIAN_POINT('Origin',(0.,-0.05953,0.));
#20381=CARTESIAN_POINT('Origin',(-0.991065754692661,-0.05953,0.477272113029314));
#20382=CARTESIAN_POINT('Origin',(-0.991065754692661,0.,0.477272113029314));
#20383=CARTESIAN_POINT('',(-1.06075609691358,-0.05953,0.181596019242328));
#20384=CARTESIAN_POINT('Ctrl Pts',(-1.06075609691358,-0.05953,0.181596019242328));
#20385=CARTESIAN_POINT('Ctrl Pts',(-1.05966202740332,-0.0925528133349865,
0.187986803072856));
#20386=CARTESIAN_POINT('Ctrl Pts',(-1.05760072925372,-0.124911173756694,
0.199872254546857));
#20387=CARTESIAN_POINT('Ctrl Pts',(-1.05146158959546,-0.177924977804098,
0.22976728653846));
#20388=CARTESIAN_POINT('Ctrl Pts',(-1.04785021111757,-0.199697230012983,
0.246078686169301));
#20389=CARTESIAN_POINT('Ctrl Pts',(-1.03846709802406,-0.237895043532788,
0.283073967563097));
#20390=CARTESIAN_POINT('Ctrl Pts',(-1.03268176429485,-0.254319232363049,
0.303755815985685));
#20391=CARTESIAN_POINT('Ctrl Pts',(-1.01919893537026,-0.28018331644634,
0.346251081972725));
#20392=CARTESIAN_POINT('Ctrl Pts',(-1.01085972381132,-0.29104845371857,
0.370184399726282));
#20393=CARTESIAN_POINT('Ctrl Pts',(-0.99154738033959,-0.30527573347708,
0.419174982698463));
#20394=CARTESIAN_POINT('Ctrl Pts',(-0.980551951791748,-0.308638795020976,
0.444223188605045));
#20395=CARTESIAN_POINT('Ctrl Pts',(-0.958671816228589,-0.308638795020976,
0.489657758261848));
#20396=CARTESIAN_POINT('Ctrl Pts',(-0.945943877838127,-0.30527573347708,
0.51387163140139));
#20397=CARTESIAN_POINT('Ctrl Pts',(-0.91968254693063,-0.29104845371857,
0.559515758398093));
#20398=CARTESIAN_POINT('Ctrl Pts',(-0.906170138993533,-0.28018331644634,
0.580957796077825));
#20399=CARTESIAN_POINT('Ctrl Pts',(-0.8813524085237,-0.254319232363049,
0.617994461173994));
#20400=CARTESIAN_POINT('Ctrl Pts',(-0.868789784891799,-0.237895043532788,
0.635412538795143));
#20401=CARTESIAN_POINT('Ctrl Pts',(-0.845715984518854,-0.199697230012983,
0.66581473268113));
#20402=CARTESIAN_POINT('Ctrl Pts',(-0.835214876415962,-0.177924977804098,
0.678808213394124));
#20403=CARTESIAN_POINT('Ctrl Pts',(-0.815669690204649,-0.124911173756694,
0.702247233627224));
#20404=CARTESIAN_POINT('Ctrl Pts',(-0.807662468433796,-0.0925528133349865,
0.711269279199861));
#20405=CARTESIAN_POINT('Ctrl Pts',(-0.803348093619616,-0.05953,0.716109245731214));
#20406=CARTESIAN_POINT('Origin',(-0.991065754692661,-0.05953,0.477272113029314));
#20407=CARTESIAN_POINT('Origin',(0.,-0.05953,0.));
#20408=CARTESIAN_POINT('',(-1.076188,-0.05953,1.31795018948079E-16));
#20409=CARTESIAN_POINT('Origin',(0.,-0.05953,0.));
#20410=CARTESIAN_POINT('',(-1.06075609691358,-0.05953,-0.181596019242328));
#20411=CARTESIAN_POINT('Origin',(0.,-0.05953,0.));
#20412=CARTESIAN_POINT('Origin',(-0.991065754692661,-0.05953,-0.477272113029314));
#20413=CARTESIAN_POINT('Origin',(-0.991065754692661,0.,-0.477272113029314));
#20414=CARTESIAN_POINT('',(-0.803348093619616,-0.05953,-0.716109245731215));
#20415=CARTESIAN_POINT('Ctrl Pts',(-0.803348093619616,-0.05953,-0.716109245731215));
#20416=CARTESIAN_POINT('Ctrl Pts',(-0.807662468433795,-0.0925528133349865,
-0.711269279199862));
#20417=CARTESIAN_POINT('Ctrl Pts',(-0.815669690204649,-0.124911173756694,
-0.702247233627224));
#20418=CARTESIAN_POINT('Ctrl Pts',(-0.835214876415962,-0.177924977804098,
-0.678808213394124));
#20419=CARTESIAN_POINT('Ctrl Pts',(-0.845715984518854,-0.199697230012983,
-0.66581473268113));
#20420=CARTESIAN_POINT('Ctrl Pts',(-0.868789784891799,-0.237895043532788,
-0.635412538795143));
#20421=CARTESIAN_POINT('Ctrl Pts',(-0.8813524085237,-0.254319232363049,
-0.617994461173994));
#20422=CARTESIAN_POINT('Ctrl Pts',(-0.906170138993533,-0.28018331644634,
-0.580957796077826));
#20423=CARTESIAN_POINT('Ctrl Pts',(-0.91968254693063,-0.29104845371857,
-0.559515758398093));
#20424=CARTESIAN_POINT('Ctrl Pts',(-0.945943877838127,-0.30527573347708,
-0.51387163140139));
#20425=CARTESIAN_POINT('Ctrl Pts',(-0.958671816228589,-0.308638795020976,
-0.489657758261848));
#20426=CARTESIAN_POINT('Ctrl Pts',(-0.980551951791748,-0.308638795020976,
-0.444223188605045));
#20427=CARTESIAN_POINT('Ctrl Pts',(-0.99154738033959,-0.30527573347708,
-0.419174982698463));
#20428=CARTESIAN_POINT('Ctrl Pts',(-1.01085972381132,-0.29104845371857,
-0.370184399726282));
#20429=CARTESIAN_POINT('Ctrl Pts',(-1.01919893537026,-0.28018331644634,
-0.346251081972725));
#20430=CARTESIAN_POINT('Ctrl Pts',(-1.03268176429485,-0.254319232363049,
-0.303755815985685));
#20431=CARTESIAN_POINT('Ctrl Pts',(-1.03846709802406,-0.237895043532788,
-0.283073967563097));
#20432=CARTESIAN_POINT('Ctrl Pts',(-1.04785021111757,-0.199697230012983,
-0.246078686169302));
#20433=CARTESIAN_POINT('Ctrl Pts',(-1.05146158959546,-0.177924977804098,
-0.229767286538461));
#20434=CARTESIAN_POINT('Ctrl Pts',(-1.05760072925372,-0.124911173756694,
-0.199872254546858));
#20435=CARTESIAN_POINT('Ctrl Pts',(-1.05966202740332,-0.0925528133349864,
-0.187986803072857));
#20436=CARTESIAN_POINT('Ctrl Pts',(-1.06075609691358,-0.05953,-0.181596019242328));
#20437=CARTESIAN_POINT('Origin',(-0.991065754692661,-0.05953,-0.477272113029314));
#20438=CARTESIAN_POINT('Origin',(0.,-0.05953,0.));
#20439=CARTESIAN_POINT('',(-0.519393123750572,-0.05953,-0.942555777842682));
#20440=CARTESIAN_POINT('Origin',(0.,-0.05953,0.));
#20441=CARTESIAN_POINT('Origin',(-0.244773027351946,-0.05953,-1.07242070340001));
#20442=CARTESIAN_POINT('Origin',(-0.244773027351946,0.,-1.07242070340001));
#20443=CARTESIAN_POINT('',(0.0589974094846125,-0.05953,-1.07456964270265));
#20444=CARTESIAN_POINT('Ctrl Pts',(0.0589974094846127,-0.05953,-1.07456964270265));
#20445=CARTESIAN_POINT('Ctrl Pts',(0.0525234025782722,-0.0925528133349865,
-1.07492508698591));
#20446=CARTESIAN_POINT('Ctrl Pts',(0.0404772621979744,-0.124911173756694,
-1.07556023164702));
#20447=CARTESIAN_POINT('Ctrl Pts',(0.0099656739833481,-0.177924977804098,
-1.07622728347683));
#20448=CARTESIAN_POINT('Ctrl Pts',(-0.00674037211528096,-0.199697230012983,
-1.07633607767727));
#20449=CARTESIAN_POINT('Ctrl Pts',(-0.044896043654098,-0.237895043532788,
-1.07542044338697));
#20450=CARTESIAN_POINT('Ctrl Pts',(-0.0663467128214644,-0.254319232363049,
-1.07438230428002));
#20451=CARTESIAN_POINT('Ctrl Pts',(-0.110776745452493,-0.28018331644634,
-1.07069360430242));
#20452=CARTESIAN_POINT('Ctrl Pts',(-0.135965654106109,-0.29104845371857,
-1.06788913840721));
#20453=CARTESIAN_POINT('Ctrl Pts',(-0.188025341585962,-0.30527573347708,
-1.05996242598502));
#20454=CARTESIAN_POINT('Ctrl Pts',(-0.214892249704082,-0.308638795020976,
-1.05481642595959));
#20455=CARTESIAN_POINT('Ctrl Pts',(-0.264056468041074,-0.308638795020976,
-1.04359501395068));
#20456=CARTESIAN_POINT('Ctrl Pts',(-0.290495481564827,-0.30527573347708,
-1.036574285215));
#20457=CARTESIAN_POINT('Ctrl Pts',(-0.340838910881557,-0.291048453718569,
-1.02112815447116));
#20458=CARTESIAN_POINT('Ctrl Pts',(-0.364750145543744,-0.28018331644634,
-1.01272583306292));
#20459=CARTESIAN_POINT('Ctrl Pts',(-0.406380688682952,-0.254319232363049,
-0.996771768218699));
#20460=CARTESIAN_POINT('Ctrl Pts',(-0.426157505475872,-0.237895043532788,
-0.988400002689705));
#20461=CARTESIAN_POINT('Ctrl Pts',(-0.460931856495794,-0.199697230012983,
-0.972669835243841));
#20462=CARTESIAN_POINT('Ctrl Pts',(-0.475936279901919,-0.177924977804098,
-0.965323333309091));
#20463=CARTESIAN_POINT('Ctrl Pts',(-0.503136848051454,-0.124911173756694,
-0.951483858396181));
#20464=CARTESIAN_POINT('Ctrl Pts',(-0.513714466572041,-0.0925528133349865,
-0.945684988399766));
#20465=CARTESIAN_POINT('Ctrl Pts',(-0.519393123750572,-0.05953,-0.942555777842682));
#20466=CARTESIAN_POINT('Origin',(-0.244773027351946,-0.05953,-1.07242070340001));
#20467=CARTESIAN_POINT('Origin',(0.,-0.05953,0.));
#20468=CARTESIAN_POINT('',(0.413083465285518,-0.05953,-0.993751811093549));
#20469=CARTESIAN_POINT('Origin',(0.,-0.05953,0.));
#20470=CARTESIAN_POINT('Origin',(0.685838782044607,-0.05953,-0.860014630714833));
#20471=CARTESIAN_POINT('Origin',(0.685838782044607,0.,-0.860014630714833));
#20472=CARTESIAN_POINT('',(0.876916659919095,-0.05953,-0.623857181492959));
#20473=CARTESIAN_POINT('Ctrl Pts',(0.876916659919095,-0.05953,-0.623857181492958));
#20474=CARTESIAN_POINT('Ctrl Pts',(0.873158080166742,-0.0925528133349865,
-0.62914037979579));
#20475=CARTESIAN_POINT('Ctrl Pts',(0.866144010579847,-0.124911173756694,
-0.638954437806245));
#20476=CARTESIAN_POINT('Ctrl Pts',(0.847641868610495,-0.177924977804098,
-0.663225258065736));
#20477=CARTESIAN_POINT('Ctrl Pts',(0.837310877969633,-0.199697230012983,
-0.676354402927683));
#20478=CARTESIAN_POINT('Ctrl Pts',(0.81280533416753,-0.237895043532788,
-0.705614819529209));
#20479=CARTESIAN_POINT('Ctrl Pts',(0.798619410861634,-0.254319232363049,
-0.721738358858166));
#20480=CARTESIAN_POINT('Ctrl Pts',(0.768033796848072,-0.28018331644634,
-0.754175290318038));
#20481=CARTESIAN_POINT('Ctrl Pts',(0.750136149454208,-0.29104845371857,
-0.772120216227122));
#20482=CARTESIAN_POINT('Ctrl Pts',(0.711480111898423,-0.30527573347708,
-0.807879894508811));
#20483=CARTESIAN_POINT('Ctrl Pts',(0.690705563850638,-0.308638795020976,
-0.825676810575913));
#20484=CARTESIAN_POINT('Ctrl Pts',(0.651278921914856,-0.308638795020976,
-0.857118508332695));
#20485=CARTESIAN_POINT('Ctrl Pts',(0.629305439856167,-0.30527573347708,
-0.873412008702649));
#20486=CARTESIAN_POINT('Ctrl Pts',(0.585840553788742,-0.29104845371857,
-0.903141581680914));
#20487=CARTESIAN_POINT('Ctrl Pts',(0.564362943424239,-0.28018331644634,
-0.916597376014514));
#20488=CARTESIAN_POINT('Ctrl Pts',(0.525933334162556,-0.254319232363049,
-0.939198248544427));
#20489=CARTESIAN_POINT('Ctrl Pts',(0.507057380724533,-0.237895043532788,
-0.949440676105255));
#20490=CARTESIAN_POINT('Ctrl Pts',(0.473077587363686,-0.199697230012983,
-0.966820759530997));
#20491=CARTESIAN_POINT('Ctrl Pts',(0.457978755888596,-0.177924977804098,
-0.973971221090534));
#20492=CARTESIAN_POINT('Ctrl Pts',(0.430199341854858,-0.124911173756694,
-0.986608710139579));
#20493=CARTESIAN_POINT('Ctrl Pts',(0.419070565453384,-0.0925528133349865,
-0.991263089003441));
#20494=CARTESIAN_POINT('Ctrl Pts',(0.413083465285518,-0.05953,-0.993751811093549));
#20495=CARTESIAN_POINT('Origin',(0.685838782044607,-0.05953,-0.860014630714833));
#20496=CARTESIAN_POINT('Origin',(0.,-0.208355,0.));
#20497=CARTESIAN_POINT('',(-1.076188,-0.35718,1.31795018948079E-16));
#20498=CARTESIAN_POINT('Origin',(0.,-0.35718,0.));
#20499=CARTESIAN_POINT('',(-1.076188,-0.208355,1.31795018948079E-16));
#20500=CARTESIAN_POINT('',(1.03449977959455,-0.05953,0.296632461748266));
#20501=CARTESIAN_POINT('Origin',(0.,-0.05953,0.));
#20502=CARTESIAN_POINT('',(1.03449977959455,-0.05953,-0.296632461748266));
#20503=CARTESIAN_POINT('Ctrl Pts',(1.03449977959455,-0.05953,0.296632461748267));
#20504=CARTESIAN_POINT('Ctrl Pts',(1.03628691421076,-0.0925528133349865,
0.290399865505497));
#20505=CARTESIAN_POINT('Ctrl Pts',(1.03958665287714,-0.124911173756694,
0.278797079997872));
#20506=CARTESIAN_POINT('Ctrl Pts',(1.0470264474309,-0.177924977804098,0.249198913998601));
#20507=CARTESIAN_POINT('Ctrl Pts',(1.05084995891418,-0.199697230012983,
0.232935932341942));
#20508=CARTESIAN_POINT('Ctrl Pts',(1.05844771715377,-0.237895043532788,
0.195533155353269));
#20509=CARTESIAN_POINT('Ctrl Pts',(1.06220882929878,-0.254319232363049,
0.17438929156337));
#20510=CARTESIAN_POINT('Ctrl Pts',(1.06849922508772,-0.28018331644634,0.130252399648131));
#20511=CARTESIAN_POINT('Ctrl Pts',(1.07137013248666,-0.29104845371857,0.105070977154072));
#20512=CARTESIAN_POINT('Ctrl Pts',(1.07522652957392,-0.30527573347708,0.0525526752791107));
#20513=CARTESIAN_POINT('Ctrl Pts',(1.076188,-0.308638795020976,0.025214283908933));
#20514=CARTESIAN_POINT('Ctrl Pts',(1.076188,-0.308638795020976,-0.025214283908933));
#20515=CARTESIAN_POINT('Ctrl Pts',(1.07522652957392,-0.30527573347708,-0.0525526752791107));
#20516=CARTESIAN_POINT('Ctrl Pts',(1.07137013248666,-0.29104845371857,-0.105070977154072));
#20517=CARTESIAN_POINT('Ctrl Pts',(1.06849922508772,-0.28018331644634,-0.130252399648131));
#20518=CARTESIAN_POINT('Ctrl Pts',(1.06220882929878,-0.254319232363049,
-0.17438929156337));
#20519=CARTESIAN_POINT('Ctrl Pts',(1.05844771715377,-0.237895043532788,
-0.195533155353269));
#20520=CARTESIAN_POINT('Ctrl Pts',(1.05084995891418,-0.199697230012983,
-0.232935932341942));
#20521=CARTESIAN_POINT('Ctrl Pts',(1.0470264474309,-0.177924977804098,-0.249198913998601));
#20522=CARTESIAN_POINT('Ctrl Pts',(1.03958665287714,-0.124911173756694,
-0.278797079997872));
#20523=CARTESIAN_POINT('Ctrl Pts',(1.03628691421076,-0.0925528133349865,
-0.290399865505497));
#20524=CARTESIAN_POINT('Ctrl Pts',(1.03449977959455,-0.05953,-0.296632461748267));
#20525=CARTESIAN_POINT('Origin',(0.,-0.05953,0.));
#20526=CARTESIAN_POINT('Origin',(0.,-0.05953,0.));
#20527=CARTESIAN_POINT('Origin',(1.1,-0.05953,0.));
#20528=CARTESIAN_POINT('Origin',(1.1,0.,0.));
#20529=CARTESIAN_POINT('Origin',(1.1,-0.05953,0.));
#20530=CARTESIAN_POINT('Origin',(0.,-0.35718,0.));
#20531=CARTESIAN_POINT('Origin',(0.,-0.05953,0.));
#57801=UNCERTAINTY_MEASURE_WITH_UNIT(LENGTH_MEASURE(0.001),#57901,
'DISTANCE_ACCURACY_VALUE',
'Maximum model space distance between geometric entities at asserted c
onnectivities');
#57841=UNCERTAINTY_MEASURE_WITH_UNIT(LENGTH_MEASURE(0.001),#57901,
'DISTANCE_ACCURACY_VALUE',
'Maximum model space distance between geometric entities at asserted c
onnectivities');
#57860=(
GEOMETRIC_REPRESENTATION_CONTEXT(3)
GLOBAL_UNCERTAINTY_ASSIGNED_CONTEXT((#57801))
GLOBAL_UNIT_ASSIGNED_CONTEXT((#57901,#57903,#57904))
REPRESENTATION_CONTEXT('','3D')
);
#57900=(
GEOMETRIC_REPRESENTATION_CONTEXT(3)
GLOBAL_UNCERTAINTY_ASSIGNED_CONTEXT((#57841))
GLOBAL_UNIT_ASSIGNED_CONTEXT((#57901,#57903,#57904))
REPRESENTATION_CONTEXT('','3D')
);
#57901=(
LENGTH_UNIT()
NAMED_UNIT(*)
SI_UNIT(.CENTI.,.METRE.)
);
#57903=(
NAMED_UNIT(*)
PLANE_ANGLE_UNIT()
SI_UNIT($,.RADIAN.)
);
#57904=(
NAMED_UNIT(*)
SI_UNIT($,.STERADIAN.)
SOLID_ANGLE_UNIT()
);
#57923=SHAPE_DEFINITION_REPRESENTATION(#57981,#58127);
#57981=PRODUCT_DEFINITION_SHAPE('',$,#58186);
#58127=SHAPE_REPRESENTATION('',(#14552),#57860);
#58167=PRODUCT_DEFINITION_CONTEXT('part definition',#58343,'design');
#58186=PRODUCT_DEFINITION('Cage','Cage',#58244,#58167);
#58244=PRODUCT_DEFINITION_FORMATION('',$,#58363);
#58343=APPLICATION_CONTEXT(
'Core Data for Automotive Mechanical Design Process');
#58344=PRODUCT_CONTEXT('part definition',#58343,'mechanical');
#58363=PRODUCT('Cage','Cage','Cage',(#58344));
#58459=COLOUR_RGB('Grey',0.48,0.52,0.57);
#58460=FILL_AREA_STYLE_COLOUR('',#58459);
#58461=FILL_AREA_STYLE('',(#58460));
#58462=SURFACE_STYLE_FILL_AREA(#58461);
#58463=SURFACE_SIDE_STYLE('',(#58462));
#58464=SURFACE_STYLE_USAGE(.BOTH.,#58463);
#58465=PRESENTATION_STYLE_ASSIGNMENT((#58464));
ENDSEC;
END-ISO-10303-21;
